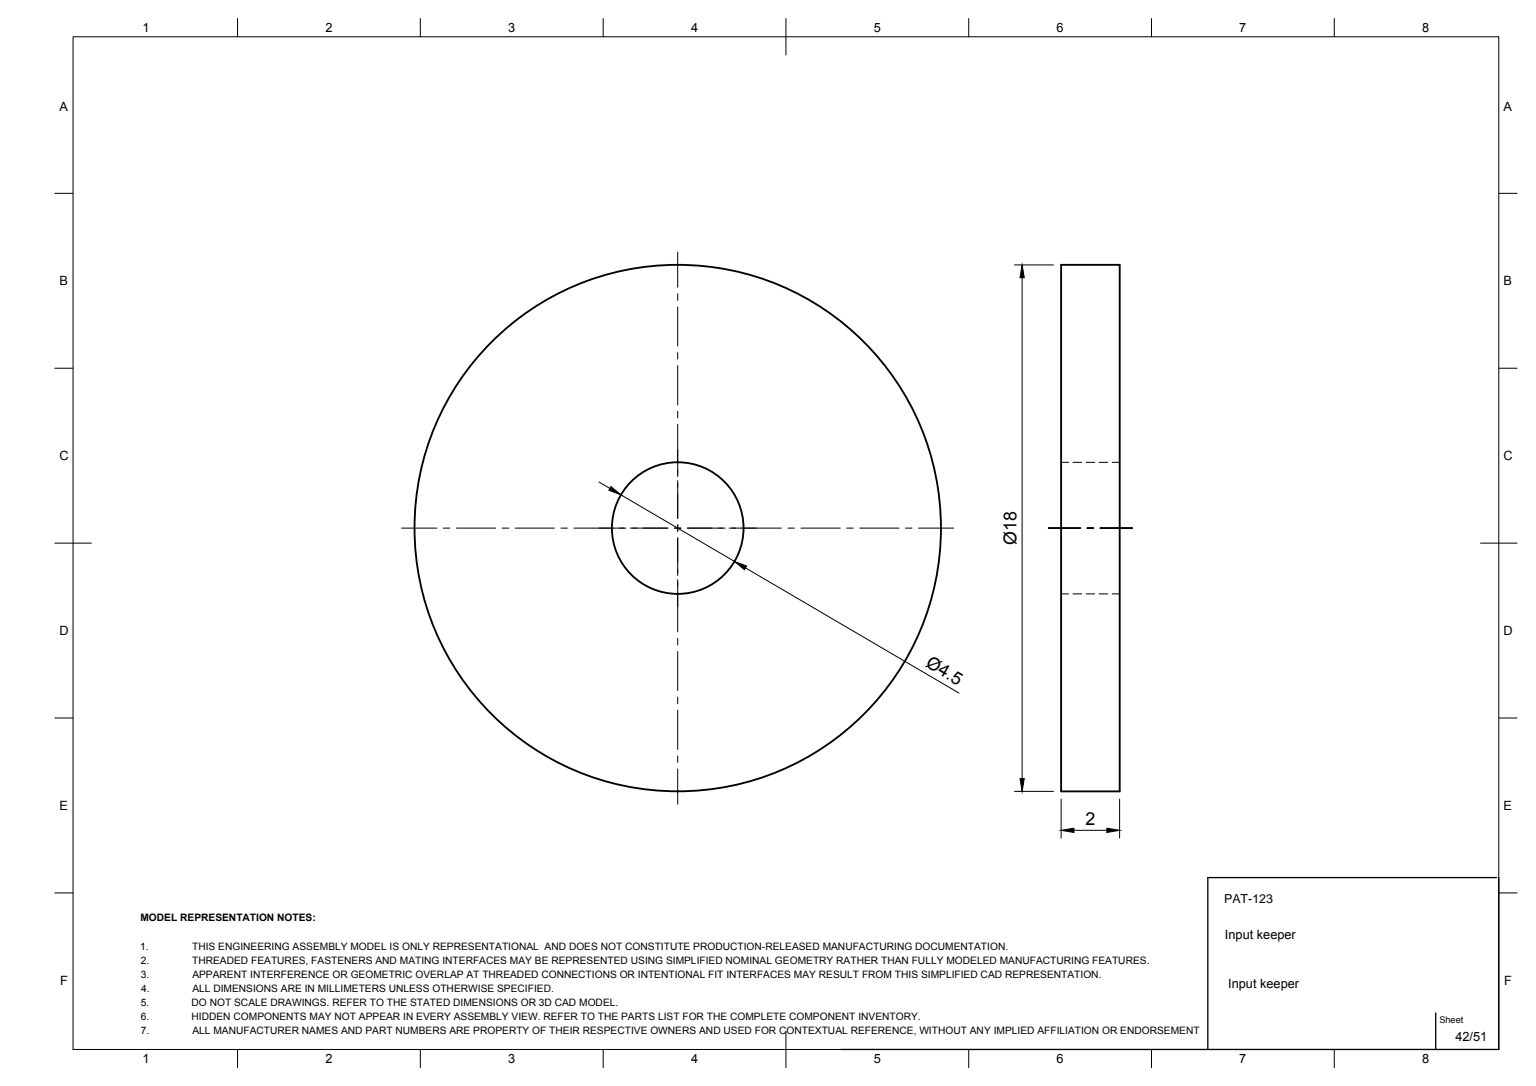
ISO-10303-21;
HEADER;
/* Generated by software containing ST-Developer
 * from STEP Tools, Inc. (www.steptools.com) 
 */

FILE_DESCRIPTION(
/* description */ ('Worm-less right-angle friction wheel drive'),
/* implementation_level */ '2;1');

FILE_NAME(
/* name */ 'Input keeper.step',
/* time_stamp */ '2026-10-28T03:22:36-07:00',
/* author */ (''),
/* organization */ (''),
/* preprocessor_version */ 'ST-DEVELOPER v20.2',
/* originating_system */ 'Autodesk Translation Framework v15.17.0.0',
/* authorisation */ '');

FILE_SCHEMA (('AUTOMOTIVE_DESIGN { 1 0 10303 214 3 1 1 }'));
ENDSEC;

DATA;
#10=MECHANICAL_DESIGN_GEOMETRIC_PRESENTATION_REPRESENTATION('',(#655),#17046);
#554=SHAPE_REPRESENTATION_RELATIONSHIP('SRR','None',#17299,#601);
#601=ADVANCED_BREP_SHAPE_REPRESENTATION('',(#706),#17035);
#655=STYLED_ITEM('',(#17605),#706);
#706=MANIFOLD_SOLID_BREP('Body1',#8213);
#934=FACE_BOUND('',#2277,.T.);
#935=FACE_BOUND('',#2279,.T.);
#1149=PLANE('',#9537);
#1150=PLANE('',#9538);
#1589=FACE_OUTER_BOUND('',#2274,.T.);
#1590=FACE_OUTER_BOUND('',#2275,.T.);
#1591=FACE_OUTER_BOUND('',#2276,.T.);
#1592=FACE_OUTER_BOUND('',#2278,.T.);
#2274=EDGE_LOOP('',(#7178,#7179,#7180,#7181));
#2275=EDGE_LOOP('',(#7182,#7183,#7184,#7185));
#2276=EDGE_LOOP('',(#7186));
#2277=EDGE_LOOP('',(#7187));
#2278=EDGE_LOOP('',(#7188));
#2279=EDGE_LOOP('',(#7189));
#2804=LINE('',#16351,#3344);
#2805=LINE('',#16357,#3345);
#3344=VECTOR('',#11782,0.225);
#3345=VECTOR('',#11789,0.9);
#3820=CIRCLE('',#9532,0.225);
#3821=CIRCLE('',#9533,0.225);
#3822=CIRCLE('',#9535,0.9);
#3823=CIRCLE('',#9536,0.9);
#4421=VERTEX_POINT('',#16348);
#4422=VERTEX_POINT('',#16350);
#4423=VERTEX_POINT('',#16354);
#4424=VERTEX_POINT('',#16356);
#5358=EDGE_CURVE('',#4421,#4421,#3820,.T.);
#5359=EDGE_CURVE('',#4421,#4422,#2804,.T.);
#5360=EDGE_CURVE('',#4422,#4422,#3821,.T.);
#5361=EDGE_CURVE('',#4423,#4423,#3822,.T.);
#5362=EDGE_CURVE('',#4423,#4424,#2805,.T.);
#5363=EDGE_CURVE('',#4424,#4424,#3823,.T.);
#7178=ORIENTED_EDGE('',*,*,#5358,.F.);
#7179=ORIENTED_EDGE('',*,*,#5359,.T.);
#7180=ORIENTED_EDGE('',*,*,#5360,.T.);
#7181=ORIENTED_EDGE('',*,*,#5359,.F.);
#7182=ORIENTED_EDGE('',*,*,#5361,.F.);
#7183=ORIENTED_EDGE('',*,*,#5362,.T.);
#7184=ORIENTED_EDGE('',*,*,#5363,.T.);
#7185=ORIENTED_EDGE('',*,*,#5362,.F.);
#7186=ORIENTED_EDGE('',*,*,#5361,.T.);
#7187=ORIENTED_EDGE('',*,*,#5358,.T.);
#7188=ORIENTED_EDGE('',*,*,#5363,.F.);
#7189=ORIENTED_EDGE('',*,*,#5360,.F.);
#7679=CYLINDRICAL_SURFACE('',#9531,0.225);
#7680=CYLINDRICAL_SURFACE('',#9534,0.9);
#8081=ADVANCED_FACE('',(#1589),#7679,.F.);
#8082=ADVANCED_FACE('',(#1590),#7680,.T.);
#8083=ADVANCED_FACE('',(#1591,#934),#1149,.T.);
#8084=ADVANCED_FACE('',(#1592,#935),#1150,.F.);
#8213=CLOSED_SHELL('',(#8081,#8082,#8083,#8084));
#9530=AXIS2_PLACEMENT_3D('',#16346,#11776,#11777);
#9531=AXIS2_PLACEMENT_3D('',#16347,#11778,#11779);
#9532=AXIS2_PLACEMENT_3D('',#16349,#11780,#11781);
#9533=AXIS2_PLACEMENT_3D('',#16352,#11783,#11784);
#9534=AXIS2_PLACEMENT_3D('',#16353,#11785,#11786);
#9535=AXIS2_PLACEMENT_3D('',#16355,#11787,#11788);
#9536=AXIS2_PLACEMENT_3D('',#16358,#11790,#11791);
#9537=AXIS2_PLACEMENT_3D('',#16359,#11792,#11793);
#9538=AXIS2_PLACEMENT_3D('',#16360,#11794,#11795);
#11776=DIRECTION('axis',(0.,0.,1.));
#11777=DIRECTION('refdir',(1.,0.,0.));
#11778=DIRECTION('center_axis',(0.,1.,0.));
#11779=DIRECTION('ref_axis',(1.,0.,0.));
#11780=DIRECTION('center_axis',(0.,-1.,0.));
#11781=DIRECTION('ref_axis',(1.,0.,0.));
#11782=DIRECTION('',(0.,-1.,0.));
#11783=DIRECTION('center_axis',(0.,-1.,0.));
#11784=DIRECTION('ref_axis',(1.,0.,0.));
#11785=DIRECTION('center_axis',(0.,1.,0.));
#11786=DIRECTION('ref_axis',(1.,0.,0.));
#11787=DIRECTION('center_axis',(0.,1.,0.));
#11788=DIRECTION('ref_axis',(1.,0.,0.));
#11789=DIRECTION('',(0.,-1.,0.));
#11790=DIRECTION('center_axis',(0.,1.,0.));
#11791=DIRECTION('ref_axis',(1.,0.,0.));
#11792=DIRECTION('center_axis',(0.,1.,0.));
#11793=DIRECTION('ref_axis',(1.,0.,0.));
#11794=DIRECTION('center_axis',(0.,1.,0.));
#11795=DIRECTION('ref_axis',(1.,0.,0.));
#16346=CARTESIAN_POINT('',(0.,0.,0.));
#16347=CARTESIAN_POINT('Origin',(0.,0.,7.));
#16348=CARTESIAN_POINT('',(-0.225,0.2,7.));
#16349=CARTESIAN_POINT('Origin',(0.,0.2,7.));
#16350=CARTESIAN_POINT('',(-0.225,0.,7.));
#16351=CARTESIAN_POINT('',(-0.225,0.,7.));
#16352=CARTESIAN_POINT('Origin',(0.,0.,7.));
#16353=CARTESIAN_POINT('Origin',(0.,0.,7.));
#16354=CARTESIAN_POINT('',(-0.9,0.2,7.));
#16355=CARTESIAN_POINT('Origin',(0.,0.2,7.));
#16356=CARTESIAN_POINT('',(-0.9,0.,7.));
#16357=CARTESIAN_POINT('',(-0.9,0.,7.));
#16358=CARTESIAN_POINT('Origin',(0.,0.,7.));
#16359=CARTESIAN_POINT('Origin',(0.,0.2,7.));
#16360=CARTESIAN_POINT('Origin',(0.,0.,7.));
#16982=UNCERTAINTY_MEASURE_WITH_UNIT(LENGTH_MEASURE(0.001),#17047,
'DISTANCE_ACCURACY_VALUE',
'Maximum model space distance between geometric entities at asserted c
onnectivities');
#16993=UNCERTAINTY_MEASURE_WITH_UNIT(LENGTH_MEASURE(0.001),#17047,
'DISTANCE_ACCURACY_VALUE',
'Maximum model space distance between geometric entities at asserted c
onnectivities');
#17035=(
GEOMETRIC_REPRESENTATION_CONTEXT(3)
GLOBAL_UNCERTAINTY_ASSIGNED_CONTEXT((#16982))
GLOBAL_UNIT_ASSIGNED_CONTEXT((#17047,#17049,#17050))
REPRESENTATION_CONTEXT('','3D')
);
#17046=(
GEOMETRIC_REPRESENTATION_CONTEXT(3)
GLOBAL_UNCERTAINTY_ASSIGNED_CONTEXT((#16993))
GLOBAL_UNIT_ASSIGNED_CONTEXT((#17047,#17049,#17050))
REPRESENTATION_CONTEXT('','3D')
);
#17047=(
LENGTH_UNIT()
NAMED_UNIT(*)
SI_UNIT(.CENTI.,.METRE.)
);
#17049=(
NAMED_UNIT(*)
PLANE_ANGLE_UNIT()
SI_UNIT($,.RADIAN.)
);
#17050=(
NAMED_UNIT(*)
SI_UNIT($,.STERADIAN.)
SOLID_ANGLE_UNIT()
);
#17092=SHAPE_DEFINITION_REPRESENTATION(#17149,#17299);
#17149=PRODUCT_DEFINITION_SHAPE('',$,#17352);
#17299=SHAPE_REPRESENTATION('',(#9530),#17035);
#17310=PRODUCT_DEFINITION_CONTEXT('part definition',#17468,'design');
#17352=PRODUCT_DEFINITION('Input keeper','Input keeper',#17404,#17310);
#17404=PRODUCT_DEFINITION_FORMATION('',$,#17511);
#17468=APPLICATION_CONTEXT(
'Core Data for Automotive Mechanical Design Process');
#17469=PRODUCT_CONTEXT('part definition',#17468,'mechanical');
#17511=PRODUCT('Input keeper','Input keeper','Input keeper',(#17469));
#17599=COLOUR_RGB('Off White',0.89,0.88,0.83);
#17600=FILL_AREA_STYLE_COLOUR('',#17599);
#17601=FILL_AREA_STYLE('',(#17600));
#17602=SURFACE_STYLE_FILL_AREA(#17601);
#17603=SURFACE_SIDE_STYLE('',(#17602));
#17604=SURFACE_STYLE_USAGE(.BOTH.,#17603);
#17605=PRESENTATION_STYLE_ASSIGNMENT((#17604));
ENDSEC;
END-ISO-10303-21;
